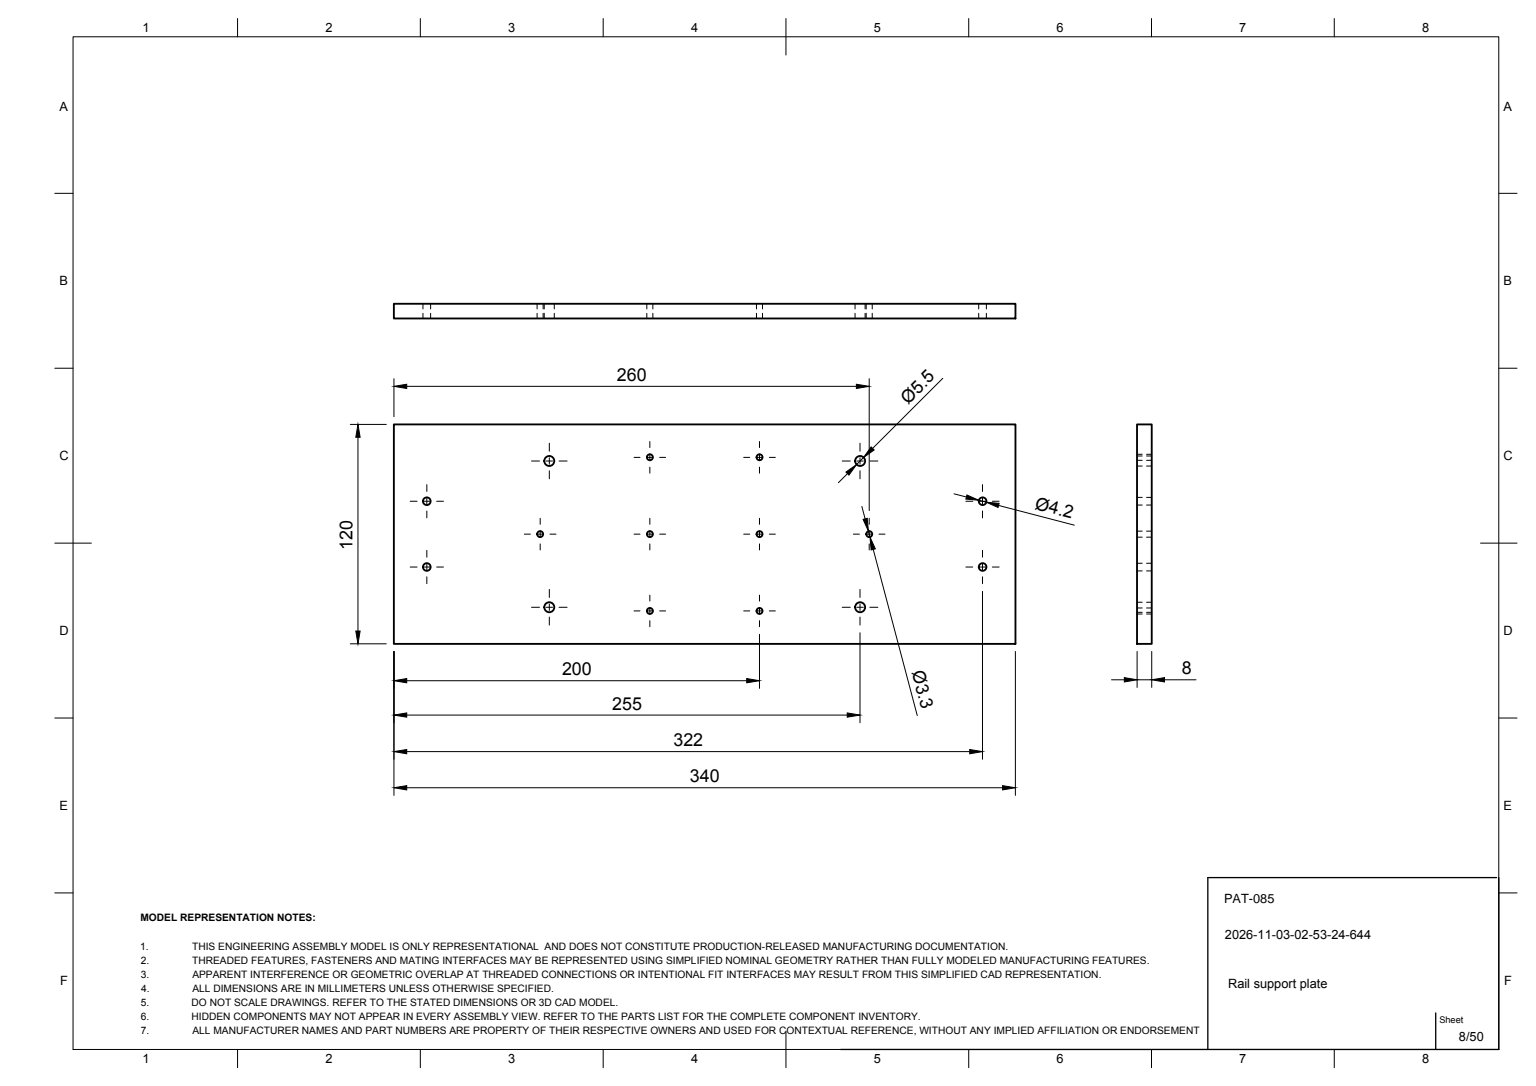
ISO-10303-21;
HEADER;
/* Generated by software containing ST-Developer
 * from STEP Tools, Inc. (www.steptools.com) 
 */

FILE_DESCRIPTION(
/* description */ ('Rack and pinion manual slide'),
/* implementation_level */ '2;1');

FILE_NAME(
/* name */ 'Rail support plate.step',
/* time_stamp */ '2026-10-28T03:22:49-07:00',
/* author */ (''),
/* organization */ (''),
/* preprocessor_version */ 'ST-DEVELOPER v20.2',
/* originating_system */ 'Autodesk Translation Framework v15.17.0.0',
/* authorisation */ '');

FILE_SCHEMA (('AUTOMOTIVE_DESIGN { 1 0 10303 214 3 1 1 }'));
ENDSEC;

DATA;
#10=MECHANICAL_DESIGN_GEOMETRIC_PRESENTATION_REPRESENTATION('',(#735),#34851);
#643=SHAPE_REPRESENTATION_RELATIONSHIP('SRR','None',#35078,#689);
#689=ADVANCED_BREP_SHAPE_REPRESENTATION('',(#788),#34803);
#735=STYLED_ITEM('',(#35425),#788);
#788=MANIFOLD_SOLID_BREP('Body1',#13755);
#841=FACE_BOUND('',#2325,.T.);
#842=FACE_BOUND('',#2326,.T.);
#843=FACE_BOUND('',#2327,.T.);
#844=FACE_BOUND('',#2328,.T.);
#845=FACE_BOUND('',#2329,.T.);
#846=FACE_BOUND('',#2330,.T.);
#847=FACE_BOUND('',#2331,.T.);
#848=FACE_BOUND('',#2332,.T.);
#849=FACE_BOUND('',#2333,.T.);
#850=FACE_BOUND('',#2334,.T.);
#851=FACE_BOUND('',#2335,.T.);
#852=FACE_BOUND('',#2336,.T.);
#853=FACE_BOUND('',#2337,.T.);
#854=FACE_BOUND('',#2338,.T.);
#855=FACE_BOUND('',#2339,.T.);
#856=FACE_BOUND('',#2340,.T.);
#857=FACE_BOUND('',#2342,.T.);
#858=FACE_BOUND('',#2343,.T.);
#859=FACE_BOUND('',#2344,.T.);
#860=FACE_BOUND('',#2345,.T.);
#861=FACE_BOUND('',#2346,.T.);
#862=FACE_BOUND('',#2347,.T.);
#863=FACE_BOUND('',#2348,.T.);
#864=FACE_BOUND('',#2349,.T.);
#865=FACE_BOUND('',#2350,.T.);
#866=FACE_BOUND('',#2351,.T.);
#867=FACE_BOUND('',#2352,.T.);
#868=FACE_BOUND('',#2353,.T.);
#869=FACE_BOUND('',#2354,.T.);
#870=FACE_BOUND('',#2355,.T.);
#871=FACE_BOUND('',#2356,.T.);
#872=FACE_BOUND('',#2357,.T.);
#1062=PLANE('',#14401);
#1063=PLANE('',#14402);
#1064=PLANE('',#14403);
#1065=PLANE('',#14404);
#1066=PLANE('',#14405);
#1067=PLANE('',#14406);
#1557=FACE_OUTER_BOUND('',#2304,.T.);
#1558=FACE_OUTER_BOUND('',#2305,.T.);
#1559=FACE_OUTER_BOUND('',#2306,.T.);
#1560=FACE_OUTER_BOUND('',#2307,.T.);
#1561=FACE_OUTER_BOUND('',#2308,.T.);
#1562=FACE_OUTER_BOUND('',#2309,.T.);
#1563=FACE_OUTER_BOUND('',#2310,.T.);
#1564=FACE_OUTER_BOUND('',#2311,.T.);
#1565=FACE_OUTER_BOUND('',#2312,.T.);
#1566=FACE_OUTER_BOUND('',#2313,.T.);
#1567=FACE_OUTER_BOUND('',#2314,.T.);
#1568=FACE_OUTER_BOUND('',#2315,.T.);
#1569=FACE_OUTER_BOUND('',#2316,.T.);
#1570=FACE_OUTER_BOUND('',#2317,.T.);
#1571=FACE_OUTER_BOUND('',#2318,.T.);
#1572=FACE_OUTER_BOUND('',#2319,.T.);
#1573=FACE_OUTER_BOUND('',#2320,.T.);
#1574=FACE_OUTER_BOUND('',#2321,.T.);
#1575=FACE_OUTER_BOUND('',#2322,.T.);
#1576=FACE_OUTER_BOUND('',#2323,.T.);
#1577=FACE_OUTER_BOUND('',#2324,.T.);
#1578=FACE_OUTER_BOUND('',#2341,.T.);
#2304=EDGE_LOOP('',(#9330,#9331,#9332,#9333));
#2305=EDGE_LOOP('',(#9334,#9335,#9336,#9337));
#2306=EDGE_LOOP('',(#9338,#9339,#9340,#9341));
#2307=EDGE_LOOP('',(#9342,#9343,#9344,#9345));
#2308=EDGE_LOOP('',(#9346,#9347,#9348,#9349));
#2309=EDGE_LOOP('',(#9350,#9351,#9352,#9353));
#2310=EDGE_LOOP('',(#9354,#9355,#9356,#9357));
#2311=EDGE_LOOP('',(#9358,#9359,#9360,#9361));
#2312=EDGE_LOOP('',(#9362,#9363,#9364,#9365));
#2313=EDGE_LOOP('',(#9366,#9367,#9368,#9369));
#2314=EDGE_LOOP('',(#9370,#9371,#9372,#9373));
#2315=EDGE_LOOP('',(#9374,#9375,#9376,#9377));
#2316=EDGE_LOOP('',(#9378,#9379,#9380,#9381));
#2317=EDGE_LOOP('',(#9382,#9383,#9384,#9385));
#2318=EDGE_LOOP('',(#9386,#9387,#9388,#9389));
#2319=EDGE_LOOP('',(#9390,#9391,#9392,#9393));
#2320=EDGE_LOOP('',(#9394,#9395,#9396,#9397));
#2321=EDGE_LOOP('',(#9398,#9399,#9400,#9401));
#2322=EDGE_LOOP('',(#9402,#9403,#9404,#9405));
#2323=EDGE_LOOP('',(#9406,#9407,#9408,#9409));
#2324=EDGE_LOOP('',(#9410,#9411,#9412,#9413));
#2325=EDGE_LOOP('',(#9414));
#2326=EDGE_LOOP('',(#9415));
#2327=EDGE_LOOP('',(#9416));
#2328=EDGE_LOOP('',(#9417));
#2329=EDGE_LOOP('',(#9418));
#2330=EDGE_LOOP('',(#9419));
#2331=EDGE_LOOP('',(#9420));
#2332=EDGE_LOOP('',(#9421));
#2333=EDGE_LOOP('',(#9422));
#2334=EDGE_LOOP('',(#9423));
#2335=EDGE_LOOP('',(#9424));
#2336=EDGE_LOOP('',(#9425));
#2337=EDGE_LOOP('',(#9426));
#2338=EDGE_LOOP('',(#9427));
#2339=EDGE_LOOP('',(#9428));
#2340=EDGE_LOOP('',(#9429));
#2341=EDGE_LOOP('',(#9430,#9431,#9432,#9433));
#2342=EDGE_LOOP('',(#9434));
#2343=EDGE_LOOP('',(#9435));
#2344=EDGE_LOOP('',(#9436));
#2345=EDGE_LOOP('',(#9437));
#2346=EDGE_LOOP('',(#9438));
#2347=EDGE_LOOP('',(#9439));
#2348=EDGE_LOOP('',(#9440));
#2349=EDGE_LOOP('',(#9441));
#2350=EDGE_LOOP('',(#9442));
#2351=EDGE_LOOP('',(#9443));
#2352=EDGE_LOOP('',(#9444));
#2353=EDGE_LOOP('',(#9445));
#2354=EDGE_LOOP('',(#9446));
#2355=EDGE_LOOP('',(#9447));
#2356=EDGE_LOOP('',(#9448));
#2357=EDGE_LOOP('',(#9449));
#3264=LINE('',#19569,#4555);
#3265=LINE('',#19575,#4556);
#3266=LINE('',#19581,#4557);
#3267=LINE('',#19587,#4558);
#3268=LINE('',#19593,#4559);
#3269=LINE('',#19599,#4560);
#3270=LINE('',#19605,#4561);
#3271=LINE('',#19611,#4562);
#3272=LINE('',#19617,#4563);
#3273=LINE('',#19623,#4564);
#3274=LINE('',#19629,#4565);
#3275=LINE('',#19635,#4566);
#3276=LINE('',#19641,#4567);
#3277=LINE('',#19647,#4568);
#3278=LINE('',#19653,#4569);
#3279=LINE('',#19659,#4570);
#3280=LINE('',#19664,#4571);
#3281=LINE('',#19666,#4572);
#3282=LINE('',#19668,#4573);
#3283=LINE('',#19669,#4574);
#3284=LINE('',#19672,#4575);
#3285=LINE('',#19674,#4576);
#3286=LINE('',#19675,#4577);
#3287=LINE('',#19678,#4578);
#3288=LINE('',#19680,#4579);
#3289=LINE('',#19681,#4580);
#3290=LINE('',#19683,#4581);
#3291=LINE('',#19684,#4582);
#4555=VECTOR('',#15716,0.164999999999999);
#4556=VECTOR('',#15723,0.164999999999999);
#4557=VECTOR('',#15730,0.164999999999999);
#4558=VECTOR('',#15737,0.164999999999999);
#4559=VECTOR('',#15744,0.210000000000001);
#4560=VECTOR('',#15751,0.210000000000001);
#4561=VECTOR('',#15758,0.21);
#4562=VECTOR('',#15765,0.21);
#4563=VECTOR('',#15772,0.164999999999999);
#4564=VECTOR('',#15779,0.164999999999999);
#4565=VECTOR('',#15786,0.165);
#4566=VECTOR('',#15793,0.164999999999999);
#4567=VECTOR('',#15800,0.274999999999999);
#4568=VECTOR('',#15807,0.274999999999999);
#4569=VECTOR('',#15814,0.275);
#4570=VECTOR('',#15821,0.275);
#4571=VECTOR('',#15826,1.);
#4572=VECTOR('',#15827,1.);
#4573=VECTOR('',#15828,1.);
#4574=VECTOR('',#15829,1.);
#4575=VECTOR('',#15832,1.);
#4576=VECTOR('',#15833,1.);
#4577=VECTOR('',#15834,1.);
#4578=VECTOR('',#15837,1.);
#4579=VECTOR('',#15838,1.);
#4580=VECTOR('',#15839,1.);
#4581=VECTOR('',#15842,1.);
#4582=VECTOR('',#15843,1.);
#5814=CIRCLE('',#14354,0.164999999999999);
#5815=CIRCLE('',#14355,0.164999999999999);
#5816=CIRCLE('',#14357,0.164999999999999);
#5817=CIRCLE('',#14358,0.164999999999999);
#5818=CIRCLE('',#14360,0.164999999999999);
#5819=CIRCLE('',#14361,0.164999999999999);
#5820=CIRCLE('',#14363,0.164999999999999);
#5821=CIRCLE('',#14364,0.164999999999999);
#5822=CIRCLE('',#14366,0.210000000000001);
#5823=CIRCLE('',#14367,0.210000000000001);
#5824=CIRCLE('',#14369,0.210000000000001);
#5825=CIRCLE('',#14370,0.210000000000001);
#5826=CIRCLE('',#14372,0.21);
#5827=CIRCLE('',#14373,0.21);
#5828=CIRCLE('',#14375,0.21);
#5829=CIRCLE('',#14376,0.21);
#5830=CIRCLE('',#14378,0.164999999999999);
#5831=CIRCLE('',#14379,0.164999999999999);
#5832=CIRCLE('',#14381,0.164999999999999);
#5833=CIRCLE('',#14382,0.164999999999999);
#5834=CIRCLE('',#14384,0.165);
#5835=CIRCLE('',#14385,0.165);
#5836=CIRCLE('',#14387,0.164999999999999);
#5837=CIRCLE('',#14388,0.164999999999999);
#5838=CIRCLE('',#14390,0.274999999999999);
#5839=CIRCLE('',#14391,0.274999999999999);
#5840=CIRCLE('',#14393,0.274999999999999);
#5841=CIRCLE('',#14394,0.274999999999999);
#5842=CIRCLE('',#14396,0.275);
#5843=CIRCLE('',#14397,0.275);
#5844=CIRCLE('',#14399,0.275);
#5845=CIRCLE('',#14400,0.275);
#6256=VERTEX_POINT('',#19566);
#6257=VERTEX_POINT('',#19568);
#6258=VERTEX_POINT('',#19572);
#6259=VERTEX_POINT('',#19574);
#6260=VERTEX_POINT('',#19578);
#6261=VERTEX_POINT('',#19580);
#6262=VERTEX_POINT('',#19584);
#6263=VERTEX_POINT('',#19586);
#6264=VERTEX_POINT('',#19590);
#6265=VERTEX_POINT('',#19592);
#6266=VERTEX_POINT('',#19596);
#6267=VERTEX_POINT('',#19598);
#6268=VERTEX_POINT('',#19602);
#6269=VERTEX_POINT('',#19604);
#6270=VERTEX_POINT('',#19608);
#6271=VERTEX_POINT('',#19610);
#6272=VERTEX_POINT('',#19614);
#6273=VERTEX_POINT('',#19616);
#6274=VERTEX_POINT('',#19620);
#6275=VERTEX_POINT('',#19622);
#6276=VERTEX_POINT('',#19626);
#6277=VERTEX_POINT('',#19628);
#6278=VERTEX_POINT('',#19632);
#6279=VERTEX_POINT('',#19634);
#6280=VERTEX_POINT('',#19638);
#6281=VERTEX_POINT('',#19640);
#6282=VERTEX_POINT('',#19644);
#6283=VERTEX_POINT('',#19646);
#6284=VERTEX_POINT('',#19650);
#6285=VERTEX_POINT('',#19652);
#6286=VERTEX_POINT('',#19656);
#6287=VERTEX_POINT('',#19658);
#6288=VERTEX_POINT('',#19662);
#6289=VERTEX_POINT('',#19663);
#6290=VERTEX_POINT('',#19665);
#6291=VERTEX_POINT('',#19667);
#6292=VERTEX_POINT('',#19671);
#6293=VERTEX_POINT('',#19673);
#6294=VERTEX_POINT('',#19677);
#6295=VERTEX_POINT('',#19679);
#7477=EDGE_CURVE('',#6256,#6256,#5814,.T.);
#7478=EDGE_CURVE('',#6256,#6257,#3264,.T.);
#7479=EDGE_CURVE('',#6257,#6257,#5815,.T.);
#7480=EDGE_CURVE('',#6258,#6258,#5816,.T.);
#7481=EDGE_CURVE('',#6258,#6259,#3265,.T.);
#7482=EDGE_CURVE('',#6259,#6259,#5817,.T.);
#7483=EDGE_CURVE('',#6260,#6260,#5818,.T.);
#7484=EDGE_CURVE('',#6260,#6261,#3266,.T.);
#7485=EDGE_CURVE('',#6261,#6261,#5819,.T.);
#7486=EDGE_CURVE('',#6262,#6262,#5820,.T.);
#7487=EDGE_CURVE('',#6262,#6263,#3267,.T.);
#7488=EDGE_CURVE('',#6263,#6263,#5821,.T.);
#7489=EDGE_CURVE('',#6264,#6264,#5822,.T.);
#7490=EDGE_CURVE('',#6264,#6265,#3268,.T.);
#7491=EDGE_CURVE('',#6265,#6265,#5823,.T.);
#7492=EDGE_CURVE('',#6266,#6266,#5824,.T.);
#7493=EDGE_CURVE('',#6266,#6267,#3269,.T.);
#7494=EDGE_CURVE('',#6267,#6267,#5825,.T.);
#7495=EDGE_CURVE('',#6268,#6268,#5826,.T.);
#7496=EDGE_CURVE('',#6268,#6269,#3270,.T.);
#7497=EDGE_CURVE('',#6269,#6269,#5827,.T.);
#7498=EDGE_CURVE('',#6270,#6270,#5828,.T.);
#7499=EDGE_CURVE('',#6270,#6271,#3271,.T.);
#7500=EDGE_CURVE('',#6271,#6271,#5829,.T.);
#7501=EDGE_CURVE('',#6272,#6272,#5830,.T.);
#7502=EDGE_CURVE('',#6272,#6273,#3272,.T.);
#7503=EDGE_CURVE('',#6273,#6273,#5831,.T.);
#7504=EDGE_CURVE('',#6274,#6274,#5832,.T.);
#7505=EDGE_CURVE('',#6274,#6275,#3273,.T.);
#7506=EDGE_CURVE('',#6275,#6275,#5833,.T.);
#7507=EDGE_CURVE('',#6276,#6276,#5834,.T.);
#7508=EDGE_CURVE('',#6276,#6277,#3274,.T.);
#7509=EDGE_CURVE('',#6277,#6277,#5835,.T.);
#7510=EDGE_CURVE('',#6278,#6278,#5836,.T.);
#7511=EDGE_CURVE('',#6278,#6279,#3275,.T.);
#7512=EDGE_CURVE('',#6279,#6279,#5837,.T.);
#7513=EDGE_CURVE('',#6280,#6280,#5838,.T.);
#7514=EDGE_CURVE('',#6280,#6281,#3276,.T.);
#7515=EDGE_CURVE('',#6281,#6281,#5839,.T.);
#7516=EDGE_CURVE('',#6282,#6282,#5840,.T.);
#7517=EDGE_CURVE('',#6282,#6283,#3277,.T.);
#7518=EDGE_CURVE('',#6283,#6283,#5841,.T.);
#7519=EDGE_CURVE('',#6284,#6284,#5842,.T.);
#7520=EDGE_CURVE('',#6284,#6285,#3278,.T.);
#7521=EDGE_CURVE('',#6285,#6285,#5843,.T.);
#7522=EDGE_CURVE('',#6286,#6286,#5844,.T.);
#7523=EDGE_CURVE('',#6286,#6287,#3279,.T.);
#7524=EDGE_CURVE('',#6287,#6287,#5845,.T.);
#7525=EDGE_CURVE('',#6288,#6289,#3280,.T.);
#7526=EDGE_CURVE('',#6289,#6290,#3281,.T.);
#7527=EDGE_CURVE('',#6291,#6290,#3282,.T.);
#7528=EDGE_CURVE('',#6288,#6291,#3283,.T.);
#7529=EDGE_CURVE('',#6292,#6288,#3284,.T.);
#7530=EDGE_CURVE('',#6293,#6291,#3285,.T.);
#7531=EDGE_CURVE('',#6292,#6293,#3286,.T.);
#7532=EDGE_CURVE('',#6294,#6292,#3287,.T.);
#7533=EDGE_CURVE('',#6295,#6293,#3288,.T.);
#7534=EDGE_CURVE('',#6294,#6295,#3289,.T.);
#7535=EDGE_CURVE('',#6289,#6294,#3290,.T.);
#7536=EDGE_CURVE('',#6290,#6295,#3291,.T.);
#9330=ORIENTED_EDGE('',*,*,#7477,.F.);
#9331=ORIENTED_EDGE('',*,*,#7478,.T.);
#9332=ORIENTED_EDGE('',*,*,#7479,.F.);
#9333=ORIENTED_EDGE('',*,*,#7478,.F.);
#9334=ORIENTED_EDGE('',*,*,#7480,.F.);
#9335=ORIENTED_EDGE('',*,*,#7481,.T.);
#9336=ORIENTED_EDGE('',*,*,#7482,.F.);
#9337=ORIENTED_EDGE('',*,*,#7481,.F.);
#9338=ORIENTED_EDGE('',*,*,#7483,.F.);
#9339=ORIENTED_EDGE('',*,*,#7484,.T.);
#9340=ORIENTED_EDGE('',*,*,#7485,.F.);
#9341=ORIENTED_EDGE('',*,*,#7484,.F.);
#9342=ORIENTED_EDGE('',*,*,#7486,.F.);
#9343=ORIENTED_EDGE('',*,*,#7487,.T.);
#9344=ORIENTED_EDGE('',*,*,#7488,.F.);
#9345=ORIENTED_EDGE('',*,*,#7487,.F.);
#9346=ORIENTED_EDGE('',*,*,#7489,.F.);
#9347=ORIENTED_EDGE('',*,*,#7490,.T.);
#9348=ORIENTED_EDGE('',*,*,#7491,.F.);
#9349=ORIENTED_EDGE('',*,*,#7490,.F.);
#9350=ORIENTED_EDGE('',*,*,#7492,.F.);
#9351=ORIENTED_EDGE('',*,*,#7493,.T.);
#9352=ORIENTED_EDGE('',*,*,#7494,.F.);
#9353=ORIENTED_EDGE('',*,*,#7493,.F.);
#9354=ORIENTED_EDGE('',*,*,#7495,.F.);
#9355=ORIENTED_EDGE('',*,*,#7496,.T.);
#9356=ORIENTED_EDGE('',*,*,#7497,.F.);
#9357=ORIENTED_EDGE('',*,*,#7496,.F.);
#9358=ORIENTED_EDGE('',*,*,#7498,.F.);
#9359=ORIENTED_EDGE('',*,*,#7499,.T.);
#9360=ORIENTED_EDGE('',*,*,#7500,.F.);
#9361=ORIENTED_EDGE('',*,*,#7499,.F.);
#9362=ORIENTED_EDGE('',*,*,#7501,.F.);
#9363=ORIENTED_EDGE('',*,*,#7502,.T.);
#9364=ORIENTED_EDGE('',*,*,#7503,.F.);
#9365=ORIENTED_EDGE('',*,*,#7502,.F.);
#9366=ORIENTED_EDGE('',*,*,#7504,.F.);
#9367=ORIENTED_EDGE('',*,*,#7505,.T.);
#9368=ORIENTED_EDGE('',*,*,#7506,.F.);
#9369=ORIENTED_EDGE('',*,*,#7505,.F.);
#9370=ORIENTED_EDGE('',*,*,#7507,.F.);
#9371=ORIENTED_EDGE('',*,*,#7508,.T.);
#9372=ORIENTED_EDGE('',*,*,#7509,.F.);
#9373=ORIENTED_EDGE('',*,*,#7508,.F.);
#9374=ORIENTED_EDGE('',*,*,#7510,.F.);
#9375=ORIENTED_EDGE('',*,*,#7511,.T.);
#9376=ORIENTED_EDGE('',*,*,#7512,.F.);
#9377=ORIENTED_EDGE('',*,*,#7511,.F.);
#9378=ORIENTED_EDGE('',*,*,#7513,.F.);
#9379=ORIENTED_EDGE('',*,*,#7514,.T.);
#9380=ORIENTED_EDGE('',*,*,#7515,.F.);
#9381=ORIENTED_EDGE('',*,*,#7514,.F.);
#9382=ORIENTED_EDGE('',*,*,#7516,.F.);
#9383=ORIENTED_EDGE('',*,*,#7517,.T.);
#9384=ORIENTED_EDGE('',*,*,#7518,.F.);
#9385=ORIENTED_EDGE('',*,*,#7517,.F.);
#9386=ORIENTED_EDGE('',*,*,#7519,.F.);
#9387=ORIENTED_EDGE('',*,*,#7520,.T.);
#9388=ORIENTED_EDGE('',*,*,#7521,.F.);
#9389=ORIENTED_EDGE('',*,*,#7520,.F.);
#9390=ORIENTED_EDGE('',*,*,#7522,.F.);
#9391=ORIENTED_EDGE('',*,*,#7523,.T.);
#9392=ORIENTED_EDGE('',*,*,#7524,.F.);
#9393=ORIENTED_EDGE('',*,*,#7523,.F.);
#9394=ORIENTED_EDGE('',*,*,#7525,.T.);
#9395=ORIENTED_EDGE('',*,*,#7526,.T.);
#9396=ORIENTED_EDGE('',*,*,#7527,.F.);
#9397=ORIENTED_EDGE('',*,*,#7528,.F.);
#9398=ORIENTED_EDGE('',*,*,#7529,.T.);
#9399=ORIENTED_EDGE('',*,*,#7528,.T.);
#9400=ORIENTED_EDGE('',*,*,#7530,.F.);
#9401=ORIENTED_EDGE('',*,*,#7531,.F.);
#9402=ORIENTED_EDGE('',*,*,#7532,.T.);
#9403=ORIENTED_EDGE('',*,*,#7531,.T.);
#9404=ORIENTED_EDGE('',*,*,#7533,.F.);
#9405=ORIENTED_EDGE('',*,*,#7534,.F.);
#9406=ORIENTED_EDGE('',*,*,#7535,.T.);
#9407=ORIENTED_EDGE('',*,*,#7534,.T.);
#9408=ORIENTED_EDGE('',*,*,#7536,.F.);
#9409=ORIENTED_EDGE('',*,*,#7526,.F.);
#9410=ORIENTED_EDGE('',*,*,#7536,.T.);
#9411=ORIENTED_EDGE('',*,*,#7533,.T.);
#9412=ORIENTED_EDGE('',*,*,#7530,.T.);
#9413=ORIENTED_EDGE('',*,*,#7527,.T.);
#9414=ORIENTED_EDGE('',*,*,#7485,.T.);
#9415=ORIENTED_EDGE('',*,*,#7488,.T.);
#9416=ORIENTED_EDGE('',*,*,#7497,.T.);
#9417=ORIENTED_EDGE('',*,*,#7500,.T.);
#9418=ORIENTED_EDGE('',*,*,#7524,.T.);
#9419=ORIENTED_EDGE('',*,*,#7521,.T.);
#9420=ORIENTED_EDGE('',*,*,#7518,.T.);
#9421=ORIENTED_EDGE('',*,*,#7515,.T.);
#9422=ORIENTED_EDGE('',*,*,#7512,.T.);
#9423=ORIENTED_EDGE('',*,*,#7509,.T.);
#9424=ORIENTED_EDGE('',*,*,#7506,.T.);
#9425=ORIENTED_EDGE('',*,*,#7503,.T.);
#9426=ORIENTED_EDGE('',*,*,#7494,.T.);
#9427=ORIENTED_EDGE('',*,*,#7491,.T.);
#9428=ORIENTED_EDGE('',*,*,#7482,.T.);
#9429=ORIENTED_EDGE('',*,*,#7479,.T.);
#9430=ORIENTED_EDGE('',*,*,#7535,.F.);
#9431=ORIENTED_EDGE('',*,*,#7525,.F.);
#9432=ORIENTED_EDGE('',*,*,#7529,.F.);
#9433=ORIENTED_EDGE('',*,*,#7532,.F.);
#9434=ORIENTED_EDGE('',*,*,#7483,.T.);
#9435=ORIENTED_EDGE('',*,*,#7486,.T.);
#9436=ORIENTED_EDGE('',*,*,#7495,.T.);
#9437=ORIENTED_EDGE('',*,*,#7498,.T.);
#9438=ORIENTED_EDGE('',*,*,#7522,.T.);
#9439=ORIENTED_EDGE('',*,*,#7519,.T.);
#9440=ORIENTED_EDGE('',*,*,#7516,.T.);
#9441=ORIENTED_EDGE('',*,*,#7513,.T.);
#9442=ORIENTED_EDGE('',*,*,#7510,.T.);
#9443=ORIENTED_EDGE('',*,*,#7507,.T.);
#9444=ORIENTED_EDGE('',*,*,#7504,.T.);
#9445=ORIENTED_EDGE('',*,*,#7501,.T.);
#9446=ORIENTED_EDGE('',*,*,#7492,.T.);
#9447=ORIENTED_EDGE('',*,*,#7489,.T.);
#9448=ORIENTED_EDGE('',*,*,#7480,.T.);
#9449=ORIENTED_EDGE('',*,*,#7477,.T.);
#12848=CYLINDRICAL_SURFACE('',#14353,0.164999999999999);
#12849=CYLINDRICAL_SURFACE('',#14356,0.164999999999999);
#12850=CYLINDRICAL_SURFACE('',#14359,0.164999999999999);
#12851=CYLINDRICAL_SURFACE('',#14362,0.164999999999999);
#12852=CYLINDRICAL_SURFACE('',#14365,0.210000000000001);
#12853=CYLINDRICAL_SURFACE('',#14368,0.210000000000001);
#12854=CYLINDRICAL_SURFACE('',#14371,0.21);
#12855=CYLINDRICAL_SURFACE('',#14374,0.21);
#12856=CYLINDRICAL_SURFACE('',#14377,0.164999999999999);
#12857=CYLINDRICAL_SURFACE('',#14380,0.164999999999999);
#12858=CYLINDRICAL_SURFACE('',#14383,0.165);
#12859=CYLINDRICAL_SURFACE('',#14386,0.164999999999999);
#12860=CYLINDRICAL_SURFACE('',#14389,0.274999999999999);
#12861=CYLINDRICAL_SURFACE('',#14392,0.274999999999999);
#12862=CYLINDRICAL_SURFACE('',#14395,0.275);
#12863=CYLINDRICAL_SURFACE('',#14398,0.275);
#13035=ADVANCED_FACE('',(#1557),#12848,.F.);
#13036=ADVANCED_FACE('',(#1558),#12849,.F.);
#13037=ADVANCED_FACE('',(#1559),#12850,.F.);
#13038=ADVANCED_FACE('',(#1560),#12851,.F.);
#13039=ADVANCED_FACE('',(#1561),#12852,.F.);
#13040=ADVANCED_FACE('',(#1562),#12853,.F.);
#13041=ADVANCED_FACE('',(#1563),#12854,.F.);
#13042=ADVANCED_FACE('',(#1564),#12855,.F.);
#13043=ADVANCED_FACE('',(#1565),#12856,.F.);
#13044=ADVANCED_FACE('',(#1566),#12857,.F.);
#13045=ADVANCED_FACE('',(#1567),#12858,.F.);
#13046=ADVANCED_FACE('',(#1568),#12859,.F.);
#13047=ADVANCED_FACE('',(#1569),#12860,.F.);
#13048=ADVANCED_FACE('',(#1570),#12861,.F.);
#13049=ADVANCED_FACE('',(#1571),#12862,.F.);
#13050=ADVANCED_FACE('',(#1572),#12863,.F.);
#13051=ADVANCED_FACE('',(#1573),#1062,.T.);
#13052=ADVANCED_FACE('',(#1574),#1063,.T.);
#13053=ADVANCED_FACE('',(#1575),#1064,.T.);
#13054=ADVANCED_FACE('',(#1576),#1065,.T.);
#13055=ADVANCED_FACE('',(#1577,#841,#842,#843,#844,#845,#846,#847,#848,
#849,#850,#851,#852,#853,#854,#855,#856),#1066,.T.);
#13056=ADVANCED_FACE('',(#1578,#857,#858,#859,#860,#861,#862,#863,#864,
#865,#866,#867,#868,#869,#870,#871,#872),#1067,.F.);
#13755=CLOSED_SHELL('',(#13035,#13036,#13037,#13038,#13039,#13040,#13041,
#13042,#13043,#13044,#13045,#13046,#13047,#13048,#13049,#13050,#13051,#13052,
#13053,#13054,#13055,#13056));
#14352=AXIS2_PLACEMENT_3D('',#19564,#15710,#15711);
#14353=AXIS2_PLACEMENT_3D('',#19565,#15712,#15713);
#14354=AXIS2_PLACEMENT_3D('',#19567,#15714,#15715);
#14355=AXIS2_PLACEMENT_3D('',#19570,#15717,#15718);
#14356=AXIS2_PLACEMENT_3D('',#19571,#15719,#15720);
#14357=AXIS2_PLACEMENT_3D('',#19573,#15721,#15722);
#14358=AXIS2_PLACEMENT_3D('',#19576,#15724,#15725);
#14359=AXIS2_PLACEMENT_3D('',#19577,#15726,#15727);
#14360=AXIS2_PLACEMENT_3D('',#19579,#15728,#15729);
#14361=AXIS2_PLACEMENT_3D('',#19582,#15731,#15732);
#14362=AXIS2_PLACEMENT_3D('',#19583,#15733,#15734);
#14363=AXIS2_PLACEMENT_3D('',#19585,#15735,#15736);
#14364=AXIS2_PLACEMENT_3D('',#19588,#15738,#15739);
#14365=AXIS2_PLACEMENT_3D('',#19589,#15740,#15741);
#14366=AXIS2_PLACEMENT_3D('',#19591,#15742,#15743);
#14367=AXIS2_PLACEMENT_3D('',#19594,#15745,#15746);
#14368=AXIS2_PLACEMENT_3D('',#19595,#15747,#15748);
#14369=AXIS2_PLACEMENT_3D('',#19597,#15749,#15750);
#14370=AXIS2_PLACEMENT_3D('',#19600,#15752,#15753);
#14371=AXIS2_PLACEMENT_3D('',#19601,#15754,#15755);
#14372=AXIS2_PLACEMENT_3D('',#19603,#15756,#15757);
#14373=AXIS2_PLACEMENT_3D('',#19606,#15759,#15760);
#14374=AXIS2_PLACEMENT_3D('',#19607,#15761,#15762);
#14375=AXIS2_PLACEMENT_3D('',#19609,#15763,#15764);
#14376=AXIS2_PLACEMENT_3D('',#19612,#15766,#15767);
#14377=AXIS2_PLACEMENT_3D('',#19613,#15768,#15769);
#14378=AXIS2_PLACEMENT_3D('',#19615,#15770,#15771);
#14379=AXIS2_PLACEMENT_3D('',#19618,#15773,#15774);
#14380=AXIS2_PLACEMENT_3D('',#19619,#15775,#15776);
#14381=AXIS2_PLACEMENT_3D('',#19621,#15777,#15778);
#14382=AXIS2_PLACEMENT_3D('',#19624,#15780,#15781);
#14383=AXIS2_PLACEMENT_3D('',#19625,#15782,#15783);
#14384=AXIS2_PLACEMENT_3D('',#19627,#15784,#15785);
#14385=AXIS2_PLACEMENT_3D('',#19630,#15787,#15788);
#14386=AXIS2_PLACEMENT_3D('',#19631,#15789,#15790);
#14387=AXIS2_PLACEMENT_3D('',#19633,#15791,#15792);
#14388=AXIS2_PLACEMENT_3D('',#19636,#15794,#15795);
#14389=AXIS2_PLACEMENT_3D('',#19637,#15796,#15797);
#14390=AXIS2_PLACEMENT_3D('',#19639,#15798,#15799);
#14391=AXIS2_PLACEMENT_3D('',#19642,#15801,#15802);
#14392=AXIS2_PLACEMENT_3D('',#19643,#15803,#15804);
#14393=AXIS2_PLACEMENT_3D('',#19645,#15805,#15806);
#14394=AXIS2_PLACEMENT_3D('',#19648,#15808,#15809);
#14395=AXIS2_PLACEMENT_3D('',#19649,#15810,#15811);
#14396=AXIS2_PLACEMENT_3D('',#19651,#15812,#15813);
#14397=AXIS2_PLACEMENT_3D('',#19654,#15815,#15816);
#14398=AXIS2_PLACEMENT_3D('',#19655,#15817,#15818);
#14399=AXIS2_PLACEMENT_3D('',#19657,#15819,#15820);
#14400=AXIS2_PLACEMENT_3D('',#19660,#15822,#15823);
#14401=AXIS2_PLACEMENT_3D('',#19661,#15824,#15825);
#14402=AXIS2_PLACEMENT_3D('',#19670,#15830,#15831);
#14403=AXIS2_PLACEMENT_3D('',#19676,#15835,#15836);
#14404=AXIS2_PLACEMENT_3D('',#19682,#15840,#15841);
#14405=AXIS2_PLACEMENT_3D('',#19685,#15844,#15845);
#14406=AXIS2_PLACEMENT_3D('',#19686,#15846,#15847);
#15710=DIRECTION('axis',(0.,0.,1.));
#15711=DIRECTION('refdir',(1.,0.,0.));
#15712=DIRECTION('center_axis',(0.,0.,1.));
#15713=DIRECTION('ref_axis',(1.,0.,0.));
#15714=DIRECTION('center_axis',(0.,0.,1.));
#15715=DIRECTION('ref_axis',(1.,0.,0.));
#15716=DIRECTION('',(0.,0.,1.));
#15717=DIRECTION('center_axis',(0.,0.,-1.));
#15718=DIRECTION('ref_axis',(1.,0.,0.));
#15719=DIRECTION('center_axis',(0.,0.,1.));
#15720=DIRECTION('ref_axis',(1.,0.,0.));
#15721=DIRECTION('center_axis',(0.,0.,1.));
#15722=DIRECTION('ref_axis',(1.,0.,0.));
#15723=DIRECTION('',(0.,0.,1.));
#15724=DIRECTION('center_axis',(0.,0.,-1.));
#15725=DIRECTION('ref_axis',(1.,0.,0.));
#15726=DIRECTION('center_axis',(0.,0.,1.));
#15727=DIRECTION('ref_axis',(1.,0.,0.));
#15728=DIRECTION('center_axis',(0.,0.,1.));
#15729=DIRECTION('ref_axis',(1.,0.,0.));
#15730=DIRECTION('',(0.,0.,1.));
#15731=DIRECTION('center_axis',(0.,0.,-1.));
#15732=DIRECTION('ref_axis',(1.,0.,0.));
#15733=DIRECTION('center_axis',(0.,0.,1.));
#15734=DIRECTION('ref_axis',(1.,0.,0.));
#15735=DIRECTION('center_axis',(0.,0.,1.));
#15736=DIRECTION('ref_axis',(1.,0.,0.));
#15737=DIRECTION('',(0.,0.,1.));
#15738=DIRECTION('center_axis',(0.,0.,-1.));
#15739=DIRECTION('ref_axis',(1.,0.,0.));
#15740=DIRECTION('center_axis',(0.,0.,1.));
#15741=DIRECTION('ref_axis',(1.,0.,0.));
#15742=DIRECTION('center_axis',(0.,0.,1.));
#15743=DIRECTION('ref_axis',(1.,0.,0.));
#15744=DIRECTION('',(0.,0.,1.));
#15745=DIRECTION('center_axis',(0.,0.,-1.));
#15746=DIRECTION('ref_axis',(1.,0.,0.));
#15747=DIRECTION('center_axis',(0.,0.,1.));
#15748=DIRECTION('ref_axis',(1.,0.,0.));
#15749=DIRECTION('center_axis',(0.,0.,1.));
#15750=DIRECTION('ref_axis',(1.,0.,0.));
#15751=DIRECTION('',(0.,0.,1.));
#15752=DIRECTION('center_axis',(0.,0.,-1.));
#15753=DIRECTION('ref_axis',(1.,0.,0.));
#15754=DIRECTION('center_axis',(0.,0.,1.));
#15755=DIRECTION('ref_axis',(1.,0.,0.));
#15756=DIRECTION('center_axis',(0.,0.,1.));
#15757=DIRECTION('ref_axis',(1.,0.,0.));
#15758=DIRECTION('',(0.,0.,1.));
#15759=DIRECTION('center_axis',(0.,0.,-1.));
#15760=DIRECTION('ref_axis',(1.,0.,0.));
#15761=DIRECTION('center_axis',(0.,0.,1.));
#15762=DIRECTION('ref_axis',(1.,0.,0.));
#15763=DIRECTION('center_axis',(0.,0.,1.));
#15764=DIRECTION('ref_axis',(1.,0.,0.));
#15765=DIRECTION('',(0.,0.,1.));
#15766=DIRECTION('center_axis',(0.,0.,-1.));
#15767=DIRECTION('ref_axis',(1.,0.,0.));
#15768=DIRECTION('center_axis',(0.,0.,1.));
#15769=DIRECTION('ref_axis',(1.,0.,0.));
#15770=DIRECTION('center_axis',(0.,0.,1.));
#15771=DIRECTION('ref_axis',(1.,0.,0.));
#15772=DIRECTION('',(0.,0.,1.));
#15773=DIRECTION('center_axis',(0.,0.,-1.));
#15774=DIRECTION('ref_axis',(1.,0.,0.));
#15775=DIRECTION('center_axis',(0.,0.,1.));
#15776=DIRECTION('ref_axis',(1.,0.,0.));
#15777=DIRECTION('center_axis',(0.,0.,1.));
#15778=DIRECTION('ref_axis',(1.,0.,0.));
#15779=DIRECTION('',(0.,0.,1.));
#15780=DIRECTION('center_axis',(0.,0.,-1.));
#15781=DIRECTION('ref_axis',(1.,0.,0.));
#15782=DIRECTION('center_axis',(0.,0.,1.));
#15783=DIRECTION('ref_axis',(1.,0.,0.));
#15784=DIRECTION('center_axis',(0.,0.,1.));
#15785=DIRECTION('ref_axis',(1.,0.,0.));
#15786=DIRECTION('',(0.,0.,1.));
#15787=DIRECTION('center_axis',(0.,0.,-1.));
#15788=DIRECTION('ref_axis',(1.,0.,0.));
#15789=DIRECTION('center_axis',(0.,0.,1.));
#15790=DIRECTION('ref_axis',(1.,0.,0.));
#15791=DIRECTION('center_axis',(0.,0.,1.));
#15792=DIRECTION('ref_axis',(1.,0.,0.));
#15793=DIRECTION('',(0.,0.,1.));
#15794=DIRECTION('center_axis',(0.,0.,-1.));
#15795=DIRECTION('ref_axis',(1.,0.,0.));
#15796=DIRECTION('center_axis',(0.,0.,1.));
#15797=DIRECTION('ref_axis',(1.,0.,0.));
#15798=DIRECTION('center_axis',(0.,0.,1.));
#15799=DIRECTION('ref_axis',(1.,0.,0.));
#15800=DIRECTION('',(0.,0.,1.));
#15801=DIRECTION('center_axis',(0.,0.,-1.));
#15802=DIRECTION('ref_axis',(1.,0.,0.));
#15803=DIRECTION('center_axis',(0.,0.,1.));
#15804=DIRECTION('ref_axis',(1.,0.,0.));
#15805=DIRECTION('center_axis',(0.,0.,1.));
#15806=DIRECTION('ref_axis',(1.,0.,0.));
#15807=DIRECTION('',(0.,0.,1.));
#15808=DIRECTION('center_axis',(0.,0.,-1.));
#15809=DIRECTION('ref_axis',(1.,0.,0.));
#15810=DIRECTION('center_axis',(0.,0.,1.));
#15811=DIRECTION('ref_axis',(1.,0.,0.));
#15812=DIRECTION('center_axis',(0.,0.,1.));
#15813=DIRECTION('ref_axis',(1.,0.,0.));
#15814=DIRECTION('',(0.,0.,1.));
#15815=DIRECTION('center_axis',(0.,0.,-1.));
#15816=DIRECTION('ref_axis',(1.,0.,0.));
#15817=DIRECTION('center_axis',(0.,0.,1.));
#15818=DIRECTION('ref_axis',(1.,0.,0.));
#15819=DIRECTION('center_axis',(0.,0.,1.));
#15820=DIRECTION('ref_axis',(1.,0.,0.));
#15821=DIRECTION('',(0.,0.,1.));
#15822=DIRECTION('center_axis',(0.,0.,-1.));
#15823=DIRECTION('ref_axis',(1.,0.,0.));
#15824=DIRECTION('center_axis',(0.,1.,0.));
#15825=DIRECTION('ref_axis',(-1.,0.,0.));
#15826=DIRECTION('',(-1.,0.,0.));
#15827=DIRECTION('',(0.,0.,1.));
#15828=DIRECTION('',(-1.,0.,0.));
#15829=DIRECTION('',(0.,0.,1.));
#15830=DIRECTION('center_axis',(1.,0.,0.));
#15831=DIRECTION('ref_axis',(0.,1.,0.));
#15832=DIRECTION('',(0.,1.,0.));
#15833=DIRECTION('',(0.,1.,0.));
#15834=DIRECTION('',(0.,0.,1.));
#15835=DIRECTION('center_axis',(0.,-1.,0.));
#15836=DIRECTION('ref_axis',(1.,0.,0.));
#15837=DIRECTION('',(1.,0.,0.));
#15838=DIRECTION('',(1.,0.,0.));
#15839=DIRECTION('',(0.,0.,1.));
#15840=DIRECTION('center_axis',(-1.,0.,0.));
#15841=DIRECTION('ref_axis',(0.,-1.,0.));
#15842=DIRECTION('',(0.,-1.,0.));
#15843=DIRECTION('',(0.,-1.,0.));
#15844=DIRECTION('center_axis',(0.,0.,1.));
#15845=DIRECTION('ref_axis',(1.,0.,0.));
#15846=DIRECTION('center_axis',(0.,0.,1.));
#15847=DIRECTION('ref_axis',(1.,0.,0.));
#19564=CARTESIAN_POINT('',(0.,0.,0.));
#19565=CARTESIAN_POINT('Origin',(8.,4.2,2.9));
#19566=CARTESIAN_POINT('',(7.835,4.2,3.));
#19567=CARTESIAN_POINT('Origin',(8.,4.2,3.));
#19568=CARTESIAN_POINT('',(7.835,4.2,3.8));
#19569=CARTESIAN_POINT('',(7.835,4.2,2.9));
#19570=CARTESIAN_POINT('Origin',(8.,4.2,3.8));
#19571=CARTESIAN_POINT('Origin',(14.,4.2,2.9));
#19572=CARTESIAN_POINT('',(13.835,4.2,3.));
#19573=CARTESIAN_POINT('Origin',(14.,4.2,3.));
#19574=CARTESIAN_POINT('',(13.835,4.2,3.8));
#19575=CARTESIAN_POINT('',(13.835,4.2,2.9));
#19576=CARTESIAN_POINT('Origin',(14.,4.2,3.8));
#19577=CARTESIAN_POINT('Origin',(8.,-4.2,2.9));
#19578=CARTESIAN_POINT('',(7.835,-4.2,3.));
#19579=CARTESIAN_POINT('Origin',(8.,-4.2,3.));
#19580=CARTESIAN_POINT('',(7.835,-4.2,3.8));
#19581=CARTESIAN_POINT('',(7.835,-4.2,2.9));
#19582=CARTESIAN_POINT('Origin',(8.,-4.2,3.8));
#19583=CARTESIAN_POINT('Origin',(14.,-4.2,2.9));
#19584=CARTESIAN_POINT('',(13.835,-4.2,3.));
#19585=CARTESIAN_POINT('Origin',(14.,-4.2,3.));
#19586=CARTESIAN_POINT('',(13.835,-4.2,3.8));
#19587=CARTESIAN_POINT('',(13.835,-4.2,2.9));
#19588=CARTESIAN_POINT('Origin',(14.,-4.2,3.8));
#19589=CARTESIAN_POINT('Origin',(26.2,-1.8,2.9));
#19590=CARTESIAN_POINT('',(25.99,-1.8,3.));
#19591=CARTESIAN_POINT('Origin',(26.2,-1.8,3.));
#19592=CARTESIAN_POINT('',(25.99,-1.8,3.8));
#19593=CARTESIAN_POINT('',(25.99,-1.8,2.9));
#19594=CARTESIAN_POINT('Origin',(26.2,-1.8,3.8));
#19595=CARTESIAN_POINT('Origin',(26.2,1.8,2.9));
#19596=CARTESIAN_POINT('',(25.99,1.8,3.));
#19597=CARTESIAN_POINT('Origin',(26.2,1.8,3.));
#19598=CARTESIAN_POINT('',(25.99,1.8,3.8));
#19599=CARTESIAN_POINT('',(25.99,1.8,2.9));
#19600=CARTESIAN_POINT('Origin',(26.2,1.8,3.8));
#19601=CARTESIAN_POINT('Origin',(-4.2,-1.8,2.9));
#19602=CARTESIAN_POINT('',(-4.41,-1.8,3.));
#19603=CARTESIAN_POINT('Origin',(-4.2,-1.8,3.));
#19604=CARTESIAN_POINT('',(-4.41,-1.8,3.8));
#19605=CARTESIAN_POINT('',(-4.41,-1.8,2.9));
#19606=CARTESIAN_POINT('Origin',(-4.2,-1.8,3.8));
#19607=CARTESIAN_POINT('Origin',(-4.2,1.8,2.9));
#19608=CARTESIAN_POINT('',(-4.41,1.8,3.));
#19609=CARTESIAN_POINT('Origin',(-4.2,1.8,3.));
#19610=CARTESIAN_POINT('',(-4.41,1.8,3.8));
#19611=CARTESIAN_POINT('',(-4.41,1.8,2.9));
#19612=CARTESIAN_POINT('Origin',(-4.2,1.8,3.8));
#19613=CARTESIAN_POINT('Origin',(14.,0.,2.9));
#19614=CARTESIAN_POINT('',(13.835,-2.02066721859312E-17,3.));
#19615=CARTESIAN_POINT('Origin',(14.,0.,3.));
#19616=CARTESIAN_POINT('',(13.835,2.02066721859312E-17,3.8));
#19617=CARTESIAN_POINT('',(13.835,-2.02066721859312E-17,2.9));
#19618=CARTESIAN_POINT('Origin',(14.,0.,3.8));
#19619=CARTESIAN_POINT('Origin',(8.,0.,2.9));
#19620=CARTESIAN_POINT('',(7.835,-2.02066721859312E-17,3.));
#19621=CARTESIAN_POINT('Origin',(8.,0.,3.));
#19622=CARTESIAN_POINT('',(7.835,2.02066721859312E-17,3.8));
#19623=CARTESIAN_POINT('',(7.835,-2.02066721859312E-17,2.9));
#19624=CARTESIAN_POINT('Origin',(8.,0.,3.8));
#19625=CARTESIAN_POINT('Origin',(2.,0.,2.9));
#19626=CARTESIAN_POINT('',(1.835,-2.02066721859313E-17,3.));
#19627=CARTESIAN_POINT('Origin',(2.,0.,3.));
#19628=CARTESIAN_POINT('',(1.835,2.02066721859313E-17,3.8));
#19629=CARTESIAN_POINT('',(1.835,-2.02066721859313E-17,2.9));
#19630=CARTESIAN_POINT('Origin',(2.,0.,3.8));
#19631=CARTESIAN_POINT('Origin',(20.,0.,2.9));
#19632=CARTESIAN_POINT('',(19.835,-2.02066721859312E-17,3.));
#19633=CARTESIAN_POINT('Origin',(20.,0.,3.));
#19634=CARTESIAN_POINT('',(19.835,2.02066721859312E-17,3.8));
#19635=CARTESIAN_POINT('',(19.835,-2.02066721859312E-17,2.9));
#19636=CARTESIAN_POINT('Origin',(20.,0.,3.8));
#19637=CARTESIAN_POINT('Origin',(19.5,4.,2.9));
#19638=CARTESIAN_POINT('',(19.225,4.,3.));
#19639=CARTESIAN_POINT('Origin',(19.5,4.,3.));
#19640=CARTESIAN_POINT('',(19.225,4.,3.8));
#19641=CARTESIAN_POINT('',(19.225,4.,2.9));
#19642=CARTESIAN_POINT('Origin',(19.5,4.,3.8));
#19643=CARTESIAN_POINT('Origin',(19.5,-4.,2.9));
#19644=CARTESIAN_POINT('',(19.225,-4.,3.));
#19645=CARTESIAN_POINT('Origin',(19.5,-4.,3.));
#19646=CARTESIAN_POINT('',(19.225,-4.,3.8));
#19647=CARTESIAN_POINT('',(19.225,-4.,2.9));
#19648=CARTESIAN_POINT('Origin',(19.5,-4.,3.8));
#19649=CARTESIAN_POINT('Origin',(2.5,4.,2.9));
#19650=CARTESIAN_POINT('',(2.225,4.,3.));
#19651=CARTESIAN_POINT('Origin',(2.5,4.,3.));
#19652=CARTESIAN_POINT('',(2.225,4.,3.8));
#19653=CARTESIAN_POINT('',(2.225,4.,2.9));
#19654=CARTESIAN_POINT('Origin',(2.5,4.,3.8));
#19655=CARTESIAN_POINT('Origin',(2.5,-4.,2.9));
#19656=CARTESIAN_POINT('',(2.225,-4.,3.));
#19657=CARTESIAN_POINT('Origin',(2.5,-4.,3.));
#19658=CARTESIAN_POINT('',(2.225,-4.,3.8));
#19659=CARTESIAN_POINT('',(2.225,-4.,2.9));
#19660=CARTESIAN_POINT('Origin',(2.5,-4.,3.8));
#19661=CARTESIAN_POINT('Origin',(28.,6.,3.));
#19662=CARTESIAN_POINT('',(28.,6.,3.));
#19663=CARTESIAN_POINT('',(-6.,6.,3.));
#19664=CARTESIAN_POINT('',(28.,6.,3.));
#19665=CARTESIAN_POINT('',(-6.,6.,3.8));
#19666=CARTESIAN_POINT('',(-6.,6.,3.));
#19667=CARTESIAN_POINT('',(28.,6.,3.8));
#19668=CARTESIAN_POINT('',(28.,6.,3.8));
#19669=CARTESIAN_POINT('',(28.,6.,3.));
#19670=CARTESIAN_POINT('Origin',(28.,-6.,3.));
#19671=CARTESIAN_POINT('',(28.,-6.,3.));
#19672=CARTESIAN_POINT('',(28.,-6.,3.));
#19673=CARTESIAN_POINT('',(28.,-6.,3.8));
#19674=CARTESIAN_POINT('',(28.,-6.,3.8));
#19675=CARTESIAN_POINT('',(28.,-6.,3.));
#19676=CARTESIAN_POINT('Origin',(-6.,-6.,3.));
#19677=CARTESIAN_POINT('',(-6.,-6.,3.));
#19678=CARTESIAN_POINT('',(-6.,-6.,3.));
#19679=CARTESIAN_POINT('',(-6.,-6.,3.8));
#19680=CARTESIAN_POINT('',(-6.,-6.,3.8));
#19681=CARTESIAN_POINT('',(-6.,-6.,3.));
#19682=CARTESIAN_POINT('Origin',(-6.,6.,3.));
#19683=CARTESIAN_POINT('',(-6.,6.,3.));
#19684=CARTESIAN_POINT('',(-6.,6.,3.8));
#19685=CARTESIAN_POINT('Origin',(11.,0.,3.8));
#19686=CARTESIAN_POINT('Origin',(11.,0.,3.));
#34749=UNCERTAINTY_MEASURE_WITH_UNIT(LENGTH_MEASURE(0.001),#34852,
'DISTANCE_ACCURACY_VALUE',
'Maximum model space distance between geometric entities at asserted c
onnectivities');
#34797=UNCERTAINTY_MEASURE_WITH_UNIT(LENGTH_MEASURE(0.001),#34852,
'DISTANCE_ACCURACY_VALUE',
'Maximum model space distance between geometric entities at asserted c
onnectivities');
#34803=(
GEOMETRIC_REPRESENTATION_CONTEXT(3)
GLOBAL_UNCERTAINTY_ASSIGNED_CONTEXT((#34749))
GLOBAL_UNIT_ASSIGNED_CONTEXT((#34852,#34854,#34855))
REPRESENTATION_CONTEXT('','3D')
);
#34851=(
GEOMETRIC_REPRESENTATION_CONTEXT(3)
GLOBAL_UNCERTAINTY_ASSIGNED_CONTEXT((#34797))
GLOBAL_UNIT_ASSIGNED_CONTEXT((#34852,#34854,#34855))
REPRESENTATION_CONTEXT('','3D')
);
#34852=(
LENGTH_UNIT()
NAMED_UNIT(*)
SI_UNIT(.CENTI.,.METRE.)
);
#34854=(
NAMED_UNIT(*)
PLANE_ANGLE_UNIT()
SI_UNIT($,.RADIAN.)
);
#34855=(
NAMED_UNIT(*)
SI_UNIT($,.STERADIAN.)
SOLID_ANGLE_UNIT()
);
#34861=SHAPE_DEFINITION_REPRESENTATION(#34914,#35078);
#34914=PRODUCT_DEFINITION_SHAPE('',$,#35132);
#35078=SHAPE_REPRESENTATION('',(#14352),#34803);
#35126=PRODUCT_DEFINITION_CONTEXT('part definition',#35287,'design');
#35132=PRODUCT_DEFINITION('Rail support plate','Rail support plate',#35185,
#35126);
#35185=PRODUCT_DEFINITION_FORMATION('',$,#35294);
#35287=APPLICATION_CONTEXT(
'Core Data for Automotive Mechanical Design Process');
#35288=PRODUCT_CONTEXT('part definition',#35287,'mechanical');
#35294=PRODUCT('Rail support plate','Rail support plate',
'Rail support plate',(#35288));
#35419=COLOUR_RGB('Off White',0.89,0.88,0.83);
#35420=FILL_AREA_STYLE_COLOUR('',#35419);
#35421=FILL_AREA_STYLE('',(#35420));
#35422=SURFACE_STYLE_FILL_AREA(#35421);
#35423=SURFACE_SIDE_STYLE('',(#35422));
#35424=SURFACE_STYLE_USAGE(.BOTH.,#35423);
#35425=PRESENTATION_STYLE_ASSIGNMENT((#35424));
ENDSEC;
END-ISO-10303-21;
